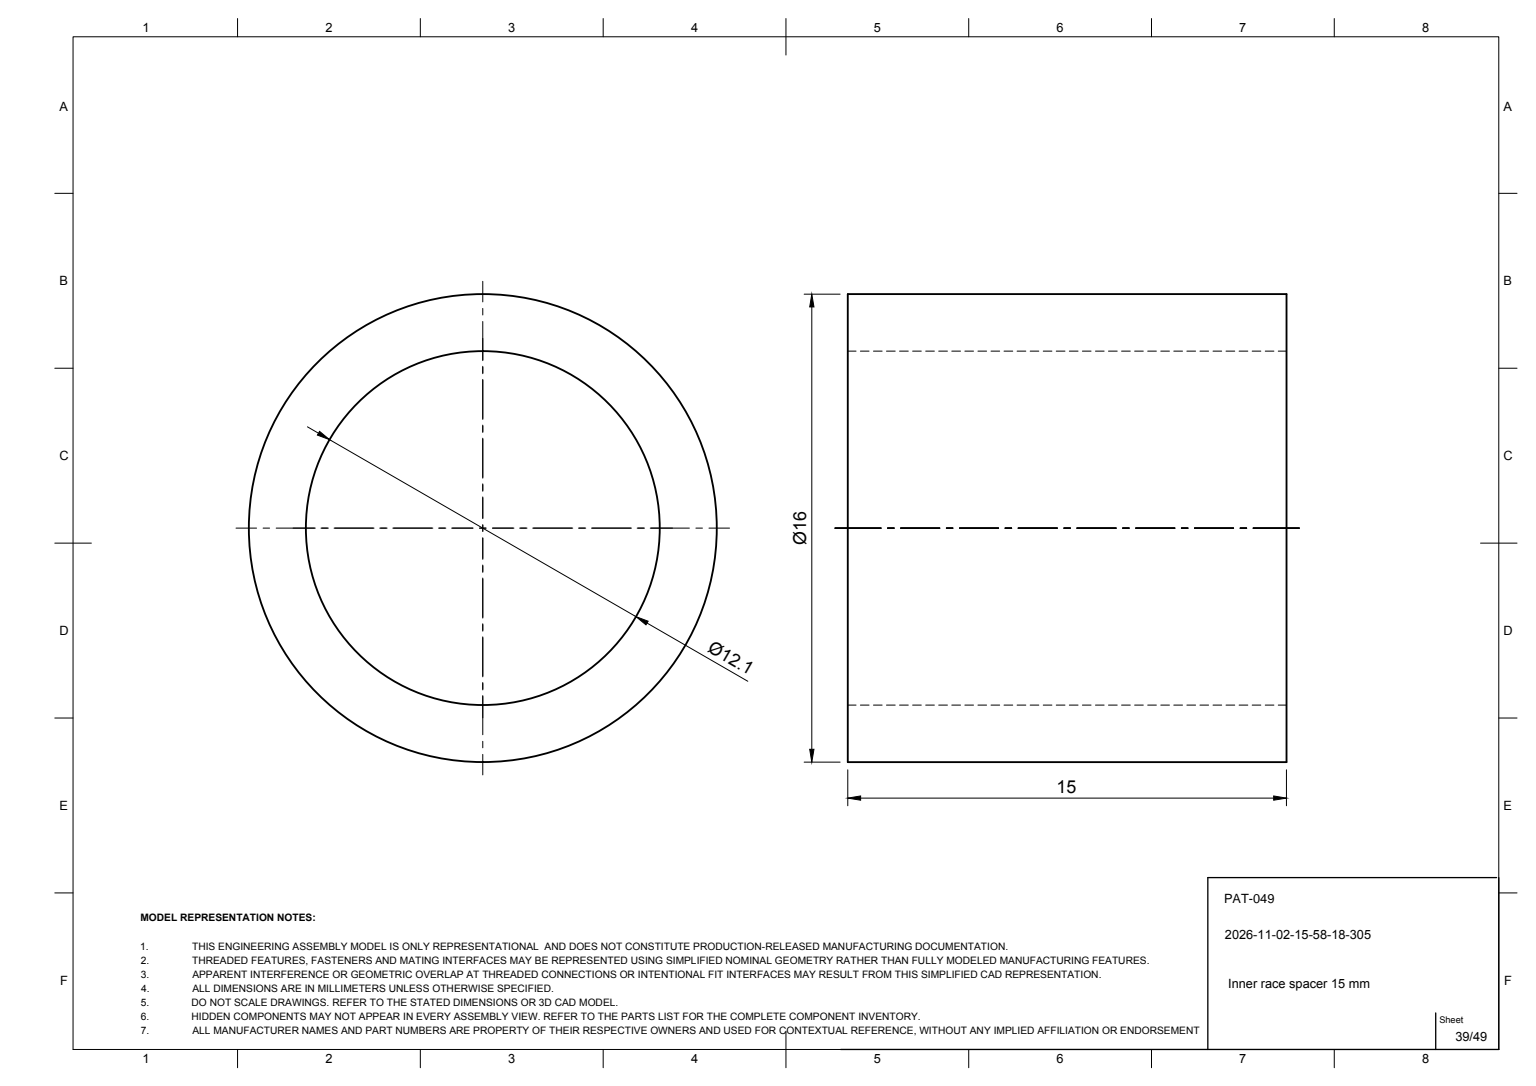
ISO-10303-21;
HEADER;
/* Generated by software containing ST-Developer
 * from STEP Tools, Inc. (www.steptools.com) 
 */

FILE_DESCRIPTION(
/* description */ ('Hand drill press frame (manual)'),
/* implementation_level */ '2;1');

FILE_NAME(
/* name */ 'Inner race spacer 15 mm.step',
/* time_stamp */ '2026-10-28T03:25:28-07:00',
/* author */ (''),
/* organization */ (''),
/* preprocessor_version */ 'ST-DEVELOPER v20.2',
/* originating_system */ 'Autodesk Translation Framework v15.17.0.0',
/* authorisation */ '');

FILE_SCHEMA (('AUTOMOTIVE_DESIGN { 1 0 10303 214 3 1 1 }'));
ENDSEC;

DATA;
#10=MECHANICAL_DESIGN_GEOMETRIC_PRESENTATION_REPRESENTATION('',(#657),#33299);
#560=SHAPE_REPRESENTATION_RELATIONSHIP('SRR','None',#33522,#605);
#605=ADVANCED_BREP_SHAPE_REPRESENTATION('',(#708),#33284);
#657=STYLED_ITEM('',(#33814),#708);
#708=MANIFOLD_SOLID_BREP('Body1',#12676);
#861=FACE_BOUND('',#2682,.T.);
#862=FACE_BOUND('',#2684,.T.);
#1254=PLANE('',#14049);
#1255=PLANE('',#14050);
#1849=FACE_OUTER_BOUND('',#2679,.T.);
#1850=FACE_OUTER_BOUND('',#2680,.T.);
#1851=FACE_OUTER_BOUND('',#2681,.T.);
#1852=FACE_OUTER_BOUND('',#2683,.T.);
#2679=EDGE_LOOP('',(#10943,#10944,#10945,#10946));
#2680=EDGE_LOOP('',(#10947,#10948,#10949,#10950));
#2681=EDGE_LOOP('',(#10951));
#2682=EDGE_LOOP('',(#10952));
#2683=EDGE_LOOP('',(#10953));
#2684=EDGE_LOOP('',(#10954));
#3810=LINE('',#21159,#4975);
#3811=LINE('',#21165,#4976);
#4975=VECTOR('',#17007,0.605);
#4976=VECTOR('',#17014,0.8);
#5511=CIRCLE('',#14044,0.605);
#5512=CIRCLE('',#14045,0.605);
#5513=CIRCLE('',#14047,0.8);
#5514=CIRCLE('',#14048,0.8);
#6461=VERTEX_POINT('',#21156);
#6462=VERTEX_POINT('',#21158);
#6463=VERTEX_POINT('',#21162);
#6464=VERTEX_POINT('',#21164);
#8000=EDGE_CURVE('',#6461,#6461,#5511,.T.);
#8001=EDGE_CURVE('',#6461,#6462,#3810,.T.);
#8002=EDGE_CURVE('',#6462,#6462,#5512,.T.);
#8003=EDGE_CURVE('',#6463,#6463,#5513,.T.);
#8004=EDGE_CURVE('',#6463,#6464,#3811,.T.);
#8005=EDGE_CURVE('',#6464,#6464,#5514,.T.);
#10943=ORIENTED_EDGE('',*,*,#8000,.F.);
#10944=ORIENTED_EDGE('',*,*,#8001,.T.);
#10945=ORIENTED_EDGE('',*,*,#8002,.T.);
#10946=ORIENTED_EDGE('',*,*,#8001,.F.);
#10947=ORIENTED_EDGE('',*,*,#8003,.F.);
#10948=ORIENTED_EDGE('',*,*,#8004,.T.);
#10949=ORIENTED_EDGE('',*,*,#8005,.T.);
#10950=ORIENTED_EDGE('',*,*,#8004,.F.);
#10951=ORIENTED_EDGE('',*,*,#8003,.T.);
#10952=ORIENTED_EDGE('',*,*,#8000,.T.);
#10953=ORIENTED_EDGE('',*,*,#8005,.F.);
#10954=ORIENTED_EDGE('',*,*,#8002,.F.);
#11902=CYLINDRICAL_SURFACE('',#14043,0.605);
#11903=CYLINDRICAL_SURFACE('',#14046,0.8);
#12458=ADVANCED_FACE('',(#1849),#11902,.F.);
#12459=ADVANCED_FACE('',(#1850),#11903,.T.);
#12460=ADVANCED_FACE('',(#1851,#861),#1254,.T.);
#12461=ADVANCED_FACE('',(#1852,#862),#1255,.F.);
#12676=CLOSED_SHELL('',(#12458,#12459,#12460,#12461));
#14042=AXIS2_PLACEMENT_3D('',#21154,#17001,#17002);
#14043=AXIS2_PLACEMENT_3D('',#21155,#17003,#17004);
#14044=AXIS2_PLACEMENT_3D('',#21157,#17005,#17006);
#14045=AXIS2_PLACEMENT_3D('',#21160,#17008,#17009);
#14046=AXIS2_PLACEMENT_3D('',#21161,#17010,#17011);
#14047=AXIS2_PLACEMENT_3D('',#21163,#17012,#17013);
#14048=AXIS2_PLACEMENT_3D('',#21166,#17015,#17016);
#14049=AXIS2_PLACEMENT_3D('',#21167,#17017,#17018);
#14050=AXIS2_PLACEMENT_3D('',#21168,#17019,#17020);
#17001=DIRECTION('axis',(0.,0.,1.));
#17002=DIRECTION('refdir',(1.,0.,0.));
#17003=DIRECTION('center_axis',(0.,1.,0.));
#17004=DIRECTION('ref_axis',(1.,0.,0.));
#17005=DIRECTION('center_axis',(0.,-1.,0.));
#17006=DIRECTION('ref_axis',(1.,0.,0.));
#17007=DIRECTION('',(0.,-1.,0.));
#17008=DIRECTION('center_axis',(0.,-1.,0.));
#17009=DIRECTION('ref_axis',(1.,0.,0.));
#17010=DIRECTION('center_axis',(0.,1.,0.));
#17011=DIRECTION('ref_axis',(1.,0.,0.));
#17012=DIRECTION('center_axis',(0.,1.,0.));
#17013=DIRECTION('ref_axis',(1.,0.,0.));
#17014=DIRECTION('',(0.,-1.,0.));
#17015=DIRECTION('center_axis',(0.,1.,0.));
#17016=DIRECTION('ref_axis',(1.,0.,0.));
#17017=DIRECTION('center_axis',(0.,1.,0.));
#17018=DIRECTION('ref_axis',(1.,0.,0.));
#17019=DIRECTION('center_axis',(0.,1.,0.));
#17020=DIRECTION('ref_axis',(1.,0.,0.));
#21154=CARTESIAN_POINT('',(0.,0.,0.));
#21155=CARTESIAN_POINT('Origin',(-3.25,-2.5,20.));
#21156=CARTESIAN_POINT('',(-3.855,-1.,20.));
#21157=CARTESIAN_POINT('Origin',(-3.25,-1.,20.));
#21158=CARTESIAN_POINT('',(-3.855,-2.5,20.));
#21159=CARTESIAN_POINT('',(-3.855,-2.5,20.));
#21160=CARTESIAN_POINT('Origin',(-3.25,-2.5,20.));
#21161=CARTESIAN_POINT('Origin',(-3.25,-2.5,20.));
#21162=CARTESIAN_POINT('',(-4.05,-1.,20.));
#21163=CARTESIAN_POINT('Origin',(-3.25,-1.,20.));
#21164=CARTESIAN_POINT('',(-4.05,-2.5,20.));
#21165=CARTESIAN_POINT('',(-4.05,-2.5,20.));
#21166=CARTESIAN_POINT('Origin',(-3.25,-2.5,20.));
#21167=CARTESIAN_POINT('Origin',(-3.25,-1.,20.));
#21168=CARTESIAN_POINT('Origin',(-3.25,-2.5,20.));
#33232=UNCERTAINTY_MEASURE_WITH_UNIT(LENGTH_MEASURE(0.001),#33300,
'DISTANCE_ACCURACY_VALUE',
'Maximum model space distance between geometric entities at asserted c
onnectivities');
#33247=UNCERTAINTY_MEASURE_WITH_UNIT(LENGTH_MEASURE(0.001),#33300,
'DISTANCE_ACCURACY_VALUE',
'Maximum model space distance between geometric entities at asserted c
onnectivities');
#33284=(
GEOMETRIC_REPRESENTATION_CONTEXT(3)
GLOBAL_UNCERTAINTY_ASSIGNED_CONTEXT((#33232))
GLOBAL_UNIT_ASSIGNED_CONTEXT((#33300,#33302,#33303))
REPRESENTATION_CONTEXT('','3D')
);
#33299=(
GEOMETRIC_REPRESENTATION_CONTEXT(3)
GLOBAL_UNCERTAINTY_ASSIGNED_CONTEXT((#33247))
GLOBAL_UNIT_ASSIGNED_CONTEXT((#33300,#33302,#33303))
REPRESENTATION_CONTEXT('','3D')
);
#33300=(
LENGTH_UNIT()
NAMED_UNIT(*)
SI_UNIT(.CENTI.,.METRE.)
);
#33302=(
NAMED_UNIT(*)
PLANE_ANGLE_UNIT()
SI_UNIT($,.RADIAN.)
);
#33303=(
NAMED_UNIT(*)
SI_UNIT($,.STERADIAN.)
SOLID_ANGLE_UNIT()
);
#33340=SHAPE_DEFINITION_REPRESENTATION(#33402,#33522);
#33402=PRODUCT_DEFINITION_SHAPE('',$,#33574);
#33522=SHAPE_REPRESENTATION('',(#14042),#33284);
#33537=PRODUCT_DEFINITION_CONTEXT('part definition',#33692,'design');
#33574=PRODUCT_DEFINITION('Inner race spacer 15 mm',
'Inner race spacer 15 mm',#33625,#33537);
#33625=PRODUCT_DEFINITION_FORMATION('',$,#33730);
#33692=APPLICATION_CONTEXT(
'Core Data for Automotive Mechanical Design Process');
#33693=PRODUCT_CONTEXT('part definition',#33692,'mechanical');
#33730=PRODUCT('Inner race spacer 15 mm','Inner race spacer 15 mm',
'Inner race spacer 15 mm',(#33693));
#33808=COLOUR_RGB('Grey',0.48,0.52,0.57);
#33809=FILL_AREA_STYLE_COLOUR('',#33808);
#33810=FILL_AREA_STYLE('',(#33809));
#33811=SURFACE_STYLE_FILL_AREA(#33810);
#33812=SURFACE_SIDE_STYLE('',(#33811));
#33813=SURFACE_STYLE_USAGE(.BOTH.,#33812);
#33814=PRESENTATION_STYLE_ASSIGNMENT((#33813));
ENDSEC;
END-ISO-10303-21;
